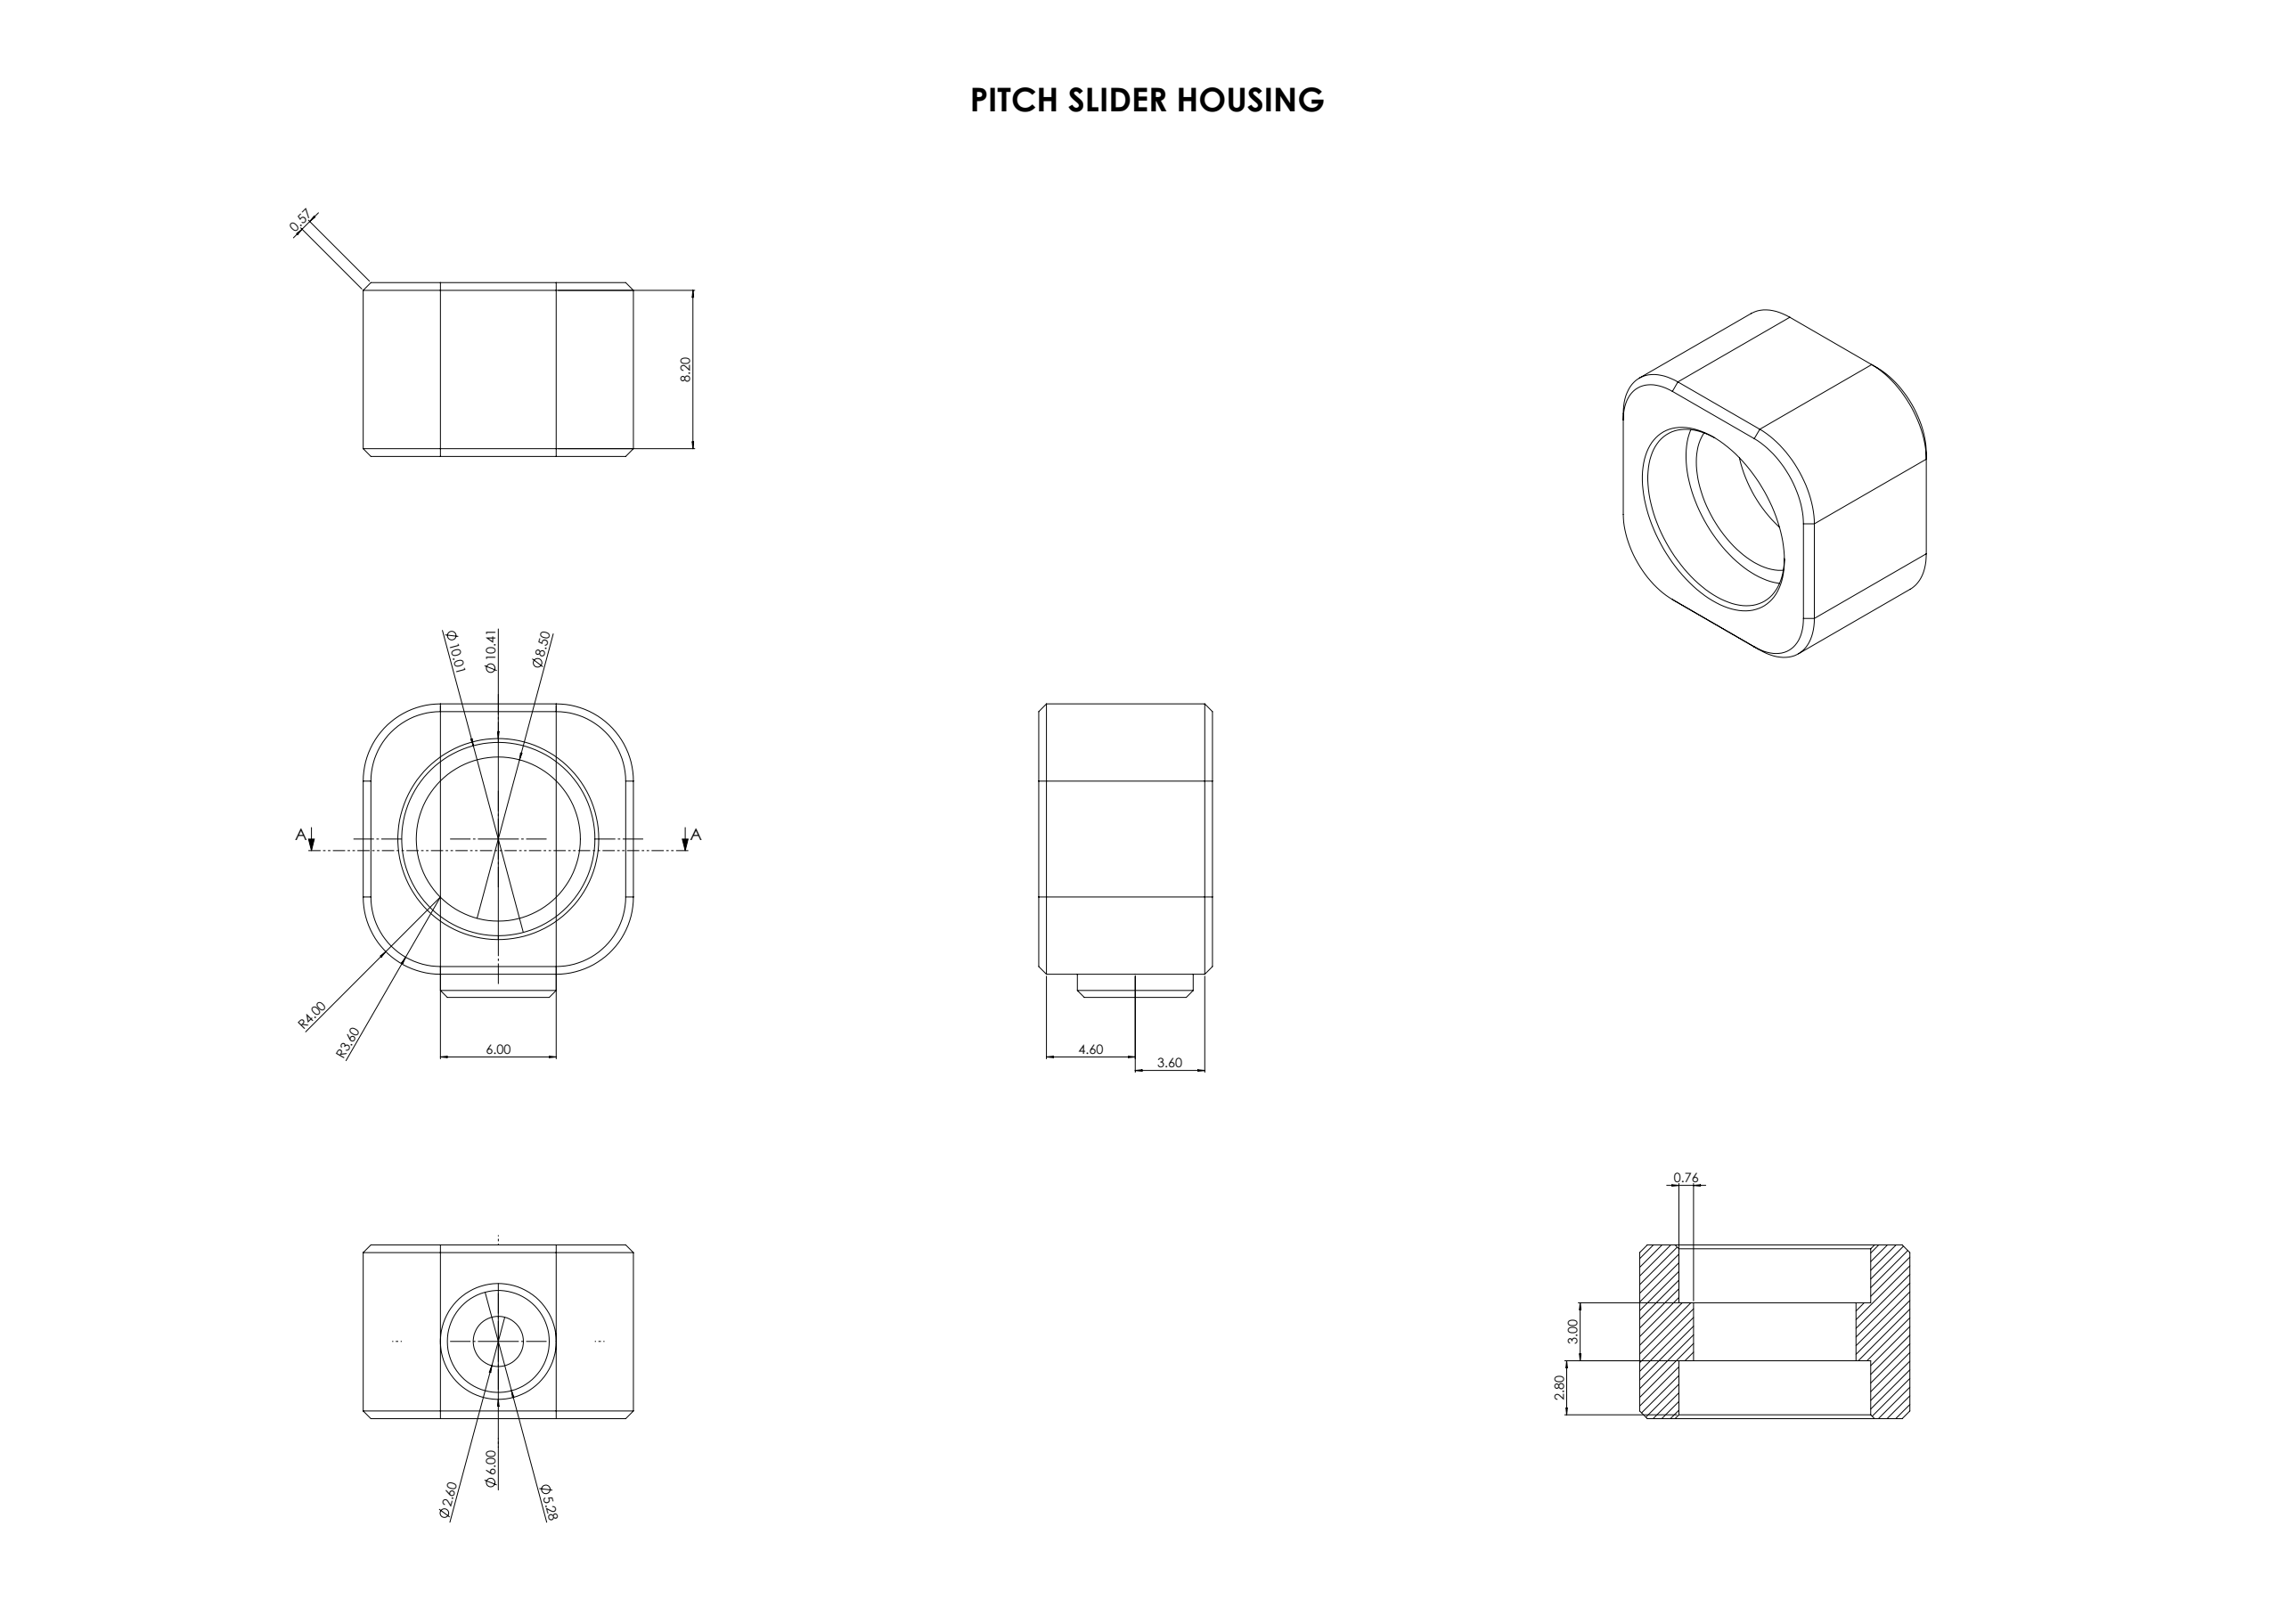
ISO-10303-21;
HEADER;
/* Generated by software containing ST-Developer
 * from STEP Tools, Inc. (www.steptools.com) 
 */

FILE_DESCRIPTION(
/* description */ (''),
/* implementation_level */ '2;1');

FILE_NAME(
/* name */ '01_Pitch_Slider_Housing.step',
/* time_stamp */ '2026-10-25T01:35:35-07:00',
/* author */ (''),
/* organization */ (''),
/* preprocessor_version */ 'ST-DEVELOPER v20.2',
/* originating_system */ 'Autodesk Translation Framework v15.15.0.0',
/* authorisation */ '');

FILE_SCHEMA (('AUTOMOTIVE_DESIGN { 1 0 10303 214 3 1 1 }'));
ENDSEC;

DATA;
#10=MECHANICAL_DESIGN_GEOMETRIC_PRESENTATION_REPRESENTATION('',(#260),#11430);
#236=SHAPE_REPRESENTATION_RELATIONSHIP('SRR','None',#11479,#248);
#248=ADVANCED_BREP_SHAPE_REPRESENTATION('',(#272),#11418);
#260=STYLED_ITEM('',(#11588),#272);
#272=MANIFOLD_SOLID_BREP('Body1',#4461);
#284=FACE_BOUND('',#797,.T.);
#285=FACE_BOUND('',#800,.T.);
#286=FACE_BOUND('',#804,.T.);
#287=FACE_BOUND('',#833,.T.);
#288=FACE_BOUND('',#836,.T.);
#323=PLANE('',#4614);
#324=PLANE('',#4619);
#325=PLANE('',#4629);
#326=PLANE('',#4636);
#327=PLANE('',#4639);
#328=PLANE('',#4642);
#329=PLANE('',#4645);
#330=PLANE('',#4650);
#331=PLANE('',#4653);
#332=PLANE('',#4654);
#333=PLANE('',#4657);
#334=PLANE('',#4660);
#335=PLANE('',#4662);
#336=PLANE('',#4665);
#337=PLANE('',#4667);
#338=PLANE('',#4670);
#339=PLANE('',#4671);
#340=PLANE('',#4675);
#341=PLANE('',#4676);
#431=CYLINDRICAL_SURFACE('',#4611,3.);
#432=CYLINDRICAL_SURFACE('',#4624,5.005);
#433=CYLINDRICAL_SURFACE('',#4634,5.005);
#434=CYLINDRICAL_SURFACE('',#4648,4.);
#435=CYLINDRICAL_SURFACE('',#4651,4.);
#436=CYLINDRICAL_SURFACE('',#4664,4.);
#437=CYLINDRICAL_SURFACE('',#4666,4.);
#438=CYLINDRICAL_SURFACE('',#4668,1.3);
#439=CYLINDRICAL_SURFACE('',#4673,4.25);
#526=FACE_OUTER_BOUND('',#794,.T.);
#527=FACE_OUTER_BOUND('',#795,.T.);
#528=FACE_OUTER_BOUND('',#796,.T.);
#529=FACE_OUTER_BOUND('',#798,.T.);
#530=FACE_OUTER_BOUND('',#799,.T.);
#531=FACE_OUTER_BOUND('',#801,.T.);
#532=FACE_OUTER_BOUND('',#802,.T.);
#533=FACE_OUTER_BOUND('',#803,.T.);
#534=FACE_OUTER_BOUND('',#805,.T.);
#535=FACE_OUTER_BOUND('',#806,.T.);
#536=FACE_OUTER_BOUND('',#807,.T.);
#537=FACE_OUTER_BOUND('',#808,.T.);
#538=FACE_OUTER_BOUND('',#809,.T.);
#539=FACE_OUTER_BOUND('',#810,.T.);
#540=FACE_OUTER_BOUND('',#811,.T.);
#541=FACE_OUTER_BOUND('',#812,.T.);
#542=FACE_OUTER_BOUND('',#813,.T.);
#543=FACE_OUTER_BOUND('',#814,.T.);
#544=FACE_OUTER_BOUND('',#815,.T.);
#545=FACE_OUTER_BOUND('',#816,.T.);
#546=FACE_OUTER_BOUND('',#817,.T.);
#547=FACE_OUTER_BOUND('',#818,.T.);
#548=FACE_OUTER_BOUND('',#819,.T.);
#549=FACE_OUTER_BOUND('',#820,.T.);
#550=FACE_OUTER_BOUND('',#821,.T.);
#551=FACE_OUTER_BOUND('',#822,.T.);
#552=FACE_OUTER_BOUND('',#823,.T.);
#553=FACE_OUTER_BOUND('',#824,.T.);
#554=FACE_OUTER_BOUND('',#825,.T.);
#555=FACE_OUTER_BOUND('',#826,.T.);
#556=FACE_OUTER_BOUND('',#827,.T.);
#557=FACE_OUTER_BOUND('',#828,.T.);
#558=FACE_OUTER_BOUND('',#829,.T.);
#559=FACE_OUTER_BOUND('',#830,.T.);
#560=FACE_OUTER_BOUND('',#831,.T.);
#561=FACE_OUTER_BOUND('',#832,.T.);
#562=FACE_OUTER_BOUND('',#834,.T.);
#563=FACE_OUTER_BOUND('',#835,.T.);
#564=FACE_OUTER_BOUND('',#837,.T.);
#794=EDGE_LOOP('',(#2885,#2886,#2887,#2888));
#795=EDGE_LOOP('',(#2889,#2890,#2891,#2892,#2893));
#796=EDGE_LOOP('',(#2894));
#797=EDGE_LOOP('',(#2895));
#798=EDGE_LOOP('',(#2896,#2897,#2898,#2899));
#799=EDGE_LOOP('',(#2900,#2901,#2902,#2903,#2904,#2905,#2906,#2907));
#800=EDGE_LOOP('',(#2908));
#801=EDGE_LOOP('',(#2909,#2910,#2911,#2912));
#802=EDGE_LOOP('',(#2913,#2914,#2915,#2916));
#803=EDGE_LOOP('',(#2917,#2918,#2919,#2920,#2921,#2922,#2923,#2924));
#804=EDGE_LOOP('',(#2925));
#805=EDGE_LOOP('',(#2926,#2927,#2928,#2929));
#806=EDGE_LOOP('',(#2930,#2931,#2932,#2933));
#807=EDGE_LOOP('',(#2934,#2935,#2936,#2937));
#808=EDGE_LOOP('',(#2938,#2939,#2940,#2941));
#809=EDGE_LOOP('',(#2942,#2943,#2944,#2945));
#810=EDGE_LOOP('',(#2946,#2947,#2948,#2949));
#811=EDGE_LOOP('',(#2950,#2951,#2952,#2953));
#812=EDGE_LOOP('',(#2954,#2955,#2956,#2957));
#813=EDGE_LOOP('',(#2958,#2959,#2960,#2961));
#814=EDGE_LOOP('',(#2962,#2963,#2964,#2965));
#815=EDGE_LOOP('',(#2966,#2967,#2968,#2969));
#816=EDGE_LOOP('',(#2970,#2971,#2972,#2973,#2974));
#817=EDGE_LOOP('',(#2975,#2976,#2977,#2978));
#818=EDGE_LOOP('',(#2979,#2980,#2981,#2982));
#819=EDGE_LOOP('',(#2983,#2984,#2985,#2986));
#820=EDGE_LOOP('',(#2987,#2988,#2989,#2990));
#821=EDGE_LOOP('',(#2991,#2992,#2993,#2994));
#822=EDGE_LOOP('',(#2995,#2996,#2997,#2998));
#823=EDGE_LOOP('',(#2999,#3000,#3001,#3002));
#824=EDGE_LOOP('',(#3003,#3004,#3005,#3006));
#825=EDGE_LOOP('',(#3007,#3008,#3009,#3010));
#826=EDGE_LOOP('',(#3011,#3012,#3013,#3014));
#827=EDGE_LOOP('',(#3015,#3016,#3017,#3018));
#828=EDGE_LOOP('',(#3019,#3020,#3021,#3022,#3023));
#829=EDGE_LOOP('',(#3024,#3025,#3026,#3027));
#830=EDGE_LOOP('',(#3028,#3029,#3030,#3031));
#831=EDGE_LOOP('',(#3032));
#832=EDGE_LOOP('',(#3033));
#833=EDGE_LOOP('',(#3034));
#834=EDGE_LOOP('',(#3035,#3036,#3037,#3038));
#835=EDGE_LOOP('',(#3039));
#836=EDGE_LOOP('',(#3040));
#837=EDGE_LOOP('',(#3041,#3042,#3043,#3044));
#1101=LINE('',#6333,#1391);
#1102=LINE('',#6337,#1392);
#1103=LINE('',#6348,#1393);
#1104=LINE('',#6353,#1394);
#1105=LINE('',#6357,#1395);
#1106=LINE('',#6361,#1396);
#1107=LINE('',#6365,#1397);
#1108=LINE('',#6370,#1398);
#1109=LINE('',#6375,#1399);
#1110=LINE('',#6380,#1400);
#1111=LINE('',#6384,#1401);
#1112=LINE('',#6388,#1402);
#1113=LINE('',#6392,#1403);
#1114=LINE('',#6396,#1404);
#1115=LINE('',#6400,#1405);
#1116=LINE('',#6402,#1406);
#1117=LINE('',#6403,#1407);
#1118=LINE('',#6406,#1408);
#1119=LINE('',#6410,#1409);
#1120=LINE('',#6411,#1410);
#1121=LINE('',#6414,#1411);
#1122=LINE('',#6418,#1412);
#1123=LINE('',#6419,#1413);
#1124=LINE('',#6422,#1414);
#1125=LINE('',#6426,#1415);
#1126=LINE('',#6427,#1416);
#1127=LINE('',#6432,#1417);
#1128=LINE('',#6435,#1418);
#1129=LINE('',#6438,#1419);
#1130=LINE('',#6439,#1420);
#1131=LINE('',#6441,#1421);
#1132=LINE('',#6443,#1422);
#1133=LINE('',#6446,#1423);
#1134=LINE('',#6449,#1424);
#1135=LINE('',#6450,#1425);
#1136=LINE('',#6451,#1426);
#1137=LINE('',#6454,#1427);
#1138=LINE('',#6458,#1428);
#1139=LINE('',#6459,#1429);
#1140=LINE('',#6462,#1430);
#1141=LINE('',#6465,#1431);
#1142=LINE('',#6466,#1432);
#1143=LINE('',#6468,#1433);
#1144=LINE('',#6470,#1434);
#1145=LINE('',#6473,#1435);
#1146=LINE('',#6474,#1436);
#1147=LINE('',#6476,#1437);
#1148=LINE('',#6478,#1438);
#1149=LINE('',#6482,#1439);
#1150=LINE('',#6490,#1440);
#1391=VECTOR('',#5091,2.82);
#1392=VECTOR('',#5096,3.);
#1393=VECTOR('',#5109,5.105);
#1394=VECTOR('',#5114,10.);
#1395=VECTOR('',#5117,10.);
#1396=VECTOR('',#5120,10.);
#1397=VECTOR('',#5123,10.);
#1398=VECTOR('',#5130,5.005);
#1399=VECTOR('',#5135,5.105);
#1400=VECTOR('',#5140,10.);
#1401=VECTOR('',#5143,10.);
#1402=VECTOR('',#5146,10.);
#1403=VECTOR('',#5149,10.);
#1404=VECTOR('',#5154,5.005);
#1405=VECTOR('',#5159,10.);
#1406=VECTOR('',#5160,10.);
#1407=VECTOR('',#5161,10.);
#1408=VECTOR('',#5164,10.);
#1409=VECTOR('',#5169,10.);
#1410=VECTOR('',#5170,10.);
#1411=VECTOR('',#5173,10.);
#1412=VECTOR('',#5178,10.);
#1413=VECTOR('',#5179,10.);
#1414=VECTOR('',#5182,10.);
#1415=VECTOR('',#5187,10.);
#1416=VECTOR('',#5188,10.);
#1417=VECTOR('',#5195,10.);
#1418=VECTOR('',#5198,10.);
#1419=VECTOR('',#5201,10.);
#1420=VECTOR('',#5202,10.);
#1421=VECTOR('',#5205,10.);
#1422=VECTOR('',#5206,10.);
#1423=VECTOR('',#5211,10.);
#1424=VECTOR('',#5214,10.);
#1425=VECTOR('',#5215,10.);
#1426=VECTOR('',#5216,10.);
#1427=VECTOR('',#5219,10.);
#1428=VECTOR('',#5224,10.);
#1429=VECTOR('',#5225,10.);
#1430=VECTOR('',#5228,10.);
#1431=VECTOR('',#5233,10.);
#1432=VECTOR('',#5234,10.);
#1433=VECTOR('',#5237,10.);
#1434=VECTOR('',#5240,10.);
#1435=VECTOR('',#5245,10.);
#1436=VECTOR('',#5246,10.);
#1437=VECTOR('',#5249,10.);
#1438=VECTOR('',#5252,10.);
#1439=VECTOR('',#5257,1.3);
#1440=VECTOR('',#5268,4.25);
#1681=CIRCLE('',#4609,2.64);
#1682=CIRCLE('',#4610,3.);
#1683=CIRCLE('',#4612,3.);
#1684=CIRCLE('',#4613,3.);
#1685=CIRCLE('',#4615,1.3);
#1686=CIRCLE('',#4617,5.205);
#1687=CIRCLE('',#4618,5.005);
#1688=CIRCLE('',#4620,3.6);
#1689=CIRCLE('',#4621,3.6);
#1690=CIRCLE('',#4622,3.6);
#1691=CIRCLE('',#4623,3.6);
#1692=CIRCLE('',#4625,5.005);
#1693=CIRCLE('',#4627,5.205);
#1694=CIRCLE('',#4628,5.005);
#1695=CIRCLE('',#4630,3.6);
#1696=CIRCLE('',#4631,3.6);
#1697=CIRCLE('',#4632,3.6);
#1698=CIRCLE('',#4633,3.6);
#1699=CIRCLE('',#4635,5.005);
#1700=CIRCLE('',#4638,4.);
#1701=CIRCLE('',#4641,4.);
#1702=CIRCLE('',#4644,4.);
#1703=CIRCLE('',#4647,4.);
#1704=CIRCLE('',#4649,4.);
#1705=CIRCLE('',#4652,4.);
#1706=CIRCLE('',#4656,4.);
#1707=CIRCLE('',#4659,4.);
#1708=CIRCLE('',#4669,1.3);
#1709=CIRCLE('',#4672,4.25);
#1710=CIRCLE('',#4674,4.25);
#1866=VERTEX_POINT('',#6330);
#1867=VERTEX_POINT('',#6332);
#1868=VERTEX_POINT('',#6336);
#1869=VERTEX_POINT('',#6338);
#1870=VERTEX_POINT('',#6342);
#1871=VERTEX_POINT('',#6345);
#1872=VERTEX_POINT('',#6347);
#1873=VERTEX_POINT('',#6351);
#1874=VERTEX_POINT('',#6352);
#1875=VERTEX_POINT('',#6354);
#1876=VERTEX_POINT('',#6356);
#1877=VERTEX_POINT('',#6358);
#1878=VERTEX_POINT('',#6360);
#1879=VERTEX_POINT('',#6362);
#1880=VERTEX_POINT('',#6364);
#1881=VERTEX_POINT('',#6368);
#1882=VERTEX_POINT('',#6372);
#1883=VERTEX_POINT('',#6374);
#1884=VERTEX_POINT('',#6378);
#1885=VERTEX_POINT('',#6379);
#1886=VERTEX_POINT('',#6381);
#1887=VERTEX_POINT('',#6383);
#1888=VERTEX_POINT('',#6385);
#1889=VERTEX_POINT('',#6387);
#1890=VERTEX_POINT('',#6389);
#1891=VERTEX_POINT('',#6391);
#1892=VERTEX_POINT('',#6395);
#1893=VERTEX_POINT('',#6399);
#1894=VERTEX_POINT('',#6401);
#1895=VERTEX_POINT('',#6405);
#1896=VERTEX_POINT('',#6409);
#1897=VERTEX_POINT('',#6413);
#1898=VERTEX_POINT('',#6417);
#1899=VERTEX_POINT('',#6421);
#1900=VERTEX_POINT('',#6425);
#1901=VERTEX_POINT('',#6431);
#1902=VERTEX_POINT('',#6433);
#1903=VERTEX_POINT('',#6437);
#1904=VERTEX_POINT('',#6442);
#1905=VERTEX_POINT('',#6448);
#1906=VERTEX_POINT('',#6453);
#1907=VERTEX_POINT('',#6457);
#1908=VERTEX_POINT('',#6461);
#1909=VERTEX_POINT('',#6481);
#1910=VERTEX_POINT('',#6486);
#1911=VERTEX_POINT('',#6489);
#2260=EDGE_CURVE('',#1866,#1866,#1681,.T.);
#2261=EDGE_CURVE('',#1866,#1867,#1101,.T.);
#2262=EDGE_CURVE('',#1867,#1867,#1682,.T.);
#2263=EDGE_CURVE('',#1867,#1868,#1102,.T.);
#2264=EDGE_CURVE('',#1869,#1868,#1683,.T.);
#2265=EDGE_CURVE('',#1868,#1869,#1684,.T.);
#2266=EDGE_CURVE('',#1870,#1870,#1685,.T.);
#2267=EDGE_CURVE('',#1871,#1871,#1686,.T.);
#2268=EDGE_CURVE('',#1871,#1872,#1103,.T.);
#2269=EDGE_CURVE('',#1872,#1872,#1687,.T.);
#2270=EDGE_CURVE('',#1873,#1874,#1104,.T.);
#2271=EDGE_CURVE('',#1875,#1873,#1688,.T.);
#2272=EDGE_CURVE('',#1876,#1875,#1105,.T.);
#2273=EDGE_CURVE('',#1877,#1876,#1689,.T.);
#2274=EDGE_CURVE('',#1878,#1877,#1106,.T.);
#2275=EDGE_CURVE('',#1879,#1878,#1690,.T.);
#2276=EDGE_CURVE('',#1880,#1879,#1107,.T.);
#2277=EDGE_CURVE('',#1874,#1880,#1691,.T.);
#2278=EDGE_CURVE('',#1881,#1881,#1692,.T.);
#2279=EDGE_CURVE('',#1881,#1872,#1108,.T.);
#2280=EDGE_CURVE('',#1882,#1882,#1693,.T.);
#2281=EDGE_CURVE('',#1882,#1883,#1109,.T.);
#2282=EDGE_CURVE('',#1883,#1883,#1694,.T.);
#2283=EDGE_CURVE('',#1884,#1885,#1110,.T.);
#2284=EDGE_CURVE('',#1886,#1884,#1695,.T.);
#2285=EDGE_CURVE('',#1887,#1886,#1111,.T.);
#2286=EDGE_CURVE('',#1888,#1887,#1696,.T.);
#2287=EDGE_CURVE('',#1889,#1888,#1112,.T.);
#2288=EDGE_CURVE('',#1890,#1889,#1697,.T.);
#2289=EDGE_CURVE('',#1891,#1890,#1113,.T.);
#2290=EDGE_CURVE('',#1885,#1891,#1698,.T.);
#2291=EDGE_CURVE('',#1883,#1892,#1114,.T.);
#2292=EDGE_CURVE('',#1892,#1892,#1699,.T.);
#2293=EDGE_CURVE('',#1885,#1893,#1115,.T.);
#2294=EDGE_CURVE('',#1893,#1894,#1116,.T.);
#2295=EDGE_CURVE('',#1894,#1884,#1117,.T.);
#2296=EDGE_CURVE('',#1891,#1895,#1118,.T.);
#2297=EDGE_CURVE('',#1895,#1893,#1700,.T.);
#2298=EDGE_CURVE('',#1890,#1896,#1119,.T.);
#2299=EDGE_CURVE('',#1896,#1895,#1120,.T.);
#2300=EDGE_CURVE('',#1889,#1897,#1121,.T.);
#2301=EDGE_CURVE('',#1897,#1896,#1701,.T.);
#2302=EDGE_CURVE('',#1888,#1898,#1122,.T.);
#2303=EDGE_CURVE('',#1898,#1897,#1123,.T.);
#2304=EDGE_CURVE('',#1887,#1899,#1124,.T.);
#2305=EDGE_CURVE('',#1899,#1898,#1702,.T.);
#2306=EDGE_CURVE('',#1886,#1900,#1125,.T.);
#2307=EDGE_CURVE('',#1900,#1899,#1126,.T.);
#2308=EDGE_CURVE('',#1894,#1900,#1703,.T.);
#2309=EDGE_CURVE('',#1899,#1901,#1127,.T.);
#2310=EDGE_CURVE('',#1902,#1901,#1704,.T.);
#2311=EDGE_CURVE('',#1898,#1902,#1128,.T.);
#2312=EDGE_CURVE('',#1900,#1903,#1129,.T.);
#2313=EDGE_CURVE('',#1901,#1903,#1130,.T.);
#2314=EDGE_CURVE('',#1894,#1868,#1131,.T.);
#2315=EDGE_CURVE('',#1868,#1904,#1132,.T.);
#2316=EDGE_CURVE('',#1903,#1904,#1705,.T.);
#2317=EDGE_CURVE('',#1893,#1869,#1133,.T.);
#2318=EDGE_CURVE('',#1905,#1873,#1134,.T.);
#2319=EDGE_CURVE('',#1874,#1904,#1135,.T.);
#2320=EDGE_CURVE('',#1904,#1905,#1136,.T.);
#2321=EDGE_CURVE('',#1906,#1875,#1137,.T.);
#2322=EDGE_CURVE('',#1905,#1906,#1706,.T.);
#2323=EDGE_CURVE('',#1907,#1876,#1138,.T.);
#2324=EDGE_CURVE('',#1906,#1907,#1139,.T.);
#2325=EDGE_CURVE('',#1908,#1877,#1140,.T.);
#2326=EDGE_CURVE('',#1907,#1908,#1707,.T.);
#2327=EDGE_CURVE('',#1902,#1878,#1141,.T.);
#2328=EDGE_CURVE('',#1908,#1902,#1142,.T.);
#2329=EDGE_CURVE('',#1901,#1879,#1143,.T.);
#2330=EDGE_CURVE('',#1903,#1880,#1144,.T.);
#2331=EDGE_CURVE('',#1897,#1908,#1145,.T.);
#2332=EDGE_CURVE('',#1896,#1907,#1146,.T.);
#2333=EDGE_CURVE('',#1895,#1906,#1147,.T.);
#2334=EDGE_CURVE('',#1869,#1905,#1148,.T.);
#2335=EDGE_CURVE('',#1870,#1909,#1149,.T.);
#2336=EDGE_CURVE('',#1909,#1909,#1708,.T.);
#2337=EDGE_CURVE('',#1910,#1910,#1709,.T.);
#2338=EDGE_CURVE('',#1910,#1911,#1150,.T.);
#2339=EDGE_CURVE('',#1911,#1911,#1710,.T.);
#2885=ORIENTED_EDGE('',*,*,#2260,.T.);
#2886=ORIENTED_EDGE('',*,*,#2261,.T.);
#2887=ORIENTED_EDGE('',*,*,#2262,.T.);
#2888=ORIENTED_EDGE('',*,*,#2261,.F.);
#2889=ORIENTED_EDGE('',*,*,#2262,.F.);
#2890=ORIENTED_EDGE('',*,*,#2263,.T.);
#2891=ORIENTED_EDGE('',*,*,#2264,.F.);
#2892=ORIENTED_EDGE('',*,*,#2265,.F.);
#2893=ORIENTED_EDGE('',*,*,#2263,.F.);
#2894=ORIENTED_EDGE('',*,*,#2260,.F.);
#2895=ORIENTED_EDGE('',*,*,#2266,.T.);
#2896=ORIENTED_EDGE('',*,*,#2267,.T.);
#2897=ORIENTED_EDGE('',*,*,#2268,.T.);
#2898=ORIENTED_EDGE('',*,*,#2269,.T.);
#2899=ORIENTED_EDGE('',*,*,#2268,.F.);
#2900=ORIENTED_EDGE('',*,*,#2270,.F.);
#2901=ORIENTED_EDGE('',*,*,#2271,.F.);
#2902=ORIENTED_EDGE('',*,*,#2272,.F.);
#2903=ORIENTED_EDGE('',*,*,#2273,.F.);
#2904=ORIENTED_EDGE('',*,*,#2274,.F.);
#2905=ORIENTED_EDGE('',*,*,#2275,.F.);
#2906=ORIENTED_EDGE('',*,*,#2276,.F.);
#2907=ORIENTED_EDGE('',*,*,#2277,.F.);
#2908=ORIENTED_EDGE('',*,*,#2267,.F.);
#2909=ORIENTED_EDGE('',*,*,#2278,.F.);
#2910=ORIENTED_EDGE('',*,*,#2279,.T.);
#2911=ORIENTED_EDGE('',*,*,#2269,.F.);
#2912=ORIENTED_EDGE('',*,*,#2279,.F.);
#2913=ORIENTED_EDGE('',*,*,#2280,.T.);
#2914=ORIENTED_EDGE('',*,*,#2281,.T.);
#2915=ORIENTED_EDGE('',*,*,#2282,.T.);
#2916=ORIENTED_EDGE('',*,*,#2281,.F.);
#2917=ORIENTED_EDGE('',*,*,#2283,.F.);
#2918=ORIENTED_EDGE('',*,*,#2284,.F.);
#2919=ORIENTED_EDGE('',*,*,#2285,.F.);
#2920=ORIENTED_EDGE('',*,*,#2286,.F.);
#2921=ORIENTED_EDGE('',*,*,#2287,.F.);
#2922=ORIENTED_EDGE('',*,*,#2288,.F.);
#2923=ORIENTED_EDGE('',*,*,#2289,.F.);
#2924=ORIENTED_EDGE('',*,*,#2290,.F.);
#2925=ORIENTED_EDGE('',*,*,#2280,.F.);
#2926=ORIENTED_EDGE('',*,*,#2282,.F.);
#2927=ORIENTED_EDGE('',*,*,#2291,.T.);
#2928=ORIENTED_EDGE('',*,*,#2292,.T.);
#2929=ORIENTED_EDGE('',*,*,#2291,.F.);
#2930=ORIENTED_EDGE('',*,*,#2293,.T.);
#2931=ORIENTED_EDGE('',*,*,#2294,.T.);
#2932=ORIENTED_EDGE('',*,*,#2295,.T.);
#2933=ORIENTED_EDGE('',*,*,#2283,.T.);
#2934=ORIENTED_EDGE('',*,*,#2296,.T.);
#2935=ORIENTED_EDGE('',*,*,#2297,.T.);
#2936=ORIENTED_EDGE('',*,*,#2293,.F.);
#2937=ORIENTED_EDGE('',*,*,#2290,.T.);
#2938=ORIENTED_EDGE('',*,*,#2298,.T.);
#2939=ORIENTED_EDGE('',*,*,#2299,.T.);
#2940=ORIENTED_EDGE('',*,*,#2296,.F.);
#2941=ORIENTED_EDGE('',*,*,#2289,.T.);
#2942=ORIENTED_EDGE('',*,*,#2300,.T.);
#2943=ORIENTED_EDGE('',*,*,#2301,.T.);
#2944=ORIENTED_EDGE('',*,*,#2298,.F.);
#2945=ORIENTED_EDGE('',*,*,#2288,.T.);
#2946=ORIENTED_EDGE('',*,*,#2302,.T.);
#2947=ORIENTED_EDGE('',*,*,#2303,.T.);
#2948=ORIENTED_EDGE('',*,*,#2300,.F.);
#2949=ORIENTED_EDGE('',*,*,#2287,.T.);
#2950=ORIENTED_EDGE('',*,*,#2304,.T.);
#2951=ORIENTED_EDGE('',*,*,#2305,.T.);
#2952=ORIENTED_EDGE('',*,*,#2302,.F.);
#2953=ORIENTED_EDGE('',*,*,#2286,.T.);
#2954=ORIENTED_EDGE('',*,*,#2306,.T.);
#2955=ORIENTED_EDGE('',*,*,#2307,.T.);
#2956=ORIENTED_EDGE('',*,*,#2304,.F.);
#2957=ORIENTED_EDGE('',*,*,#2285,.T.);
#2958=ORIENTED_EDGE('',*,*,#2295,.F.);
#2959=ORIENTED_EDGE('',*,*,#2308,.T.);
#2960=ORIENTED_EDGE('',*,*,#2306,.F.);
#2961=ORIENTED_EDGE('',*,*,#2284,.T.);
#2962=ORIENTED_EDGE('',*,*,#2305,.F.);
#2963=ORIENTED_EDGE('',*,*,#2309,.T.);
#2964=ORIENTED_EDGE('',*,*,#2310,.F.);
#2965=ORIENTED_EDGE('',*,*,#2311,.F.);
#2966=ORIENTED_EDGE('',*,*,#2307,.F.);
#2967=ORIENTED_EDGE('',*,*,#2312,.T.);
#2968=ORIENTED_EDGE('',*,*,#2313,.F.);
#2969=ORIENTED_EDGE('',*,*,#2309,.F.);
#2970=ORIENTED_EDGE('',*,*,#2308,.F.);
#2971=ORIENTED_EDGE('',*,*,#2314,.T.);
#2972=ORIENTED_EDGE('',*,*,#2315,.T.);
#2973=ORIENTED_EDGE('',*,*,#2316,.F.);
#2974=ORIENTED_EDGE('',*,*,#2312,.F.);
#2975=ORIENTED_EDGE('',*,*,#2294,.F.);
#2976=ORIENTED_EDGE('',*,*,#2317,.T.);
#2977=ORIENTED_EDGE('',*,*,#2264,.T.);
#2978=ORIENTED_EDGE('',*,*,#2314,.F.);
#2979=ORIENTED_EDGE('',*,*,#2318,.T.);
#2980=ORIENTED_EDGE('',*,*,#2270,.T.);
#2981=ORIENTED_EDGE('',*,*,#2319,.T.);
#2982=ORIENTED_EDGE('',*,*,#2320,.T.);
#2983=ORIENTED_EDGE('',*,*,#2321,.T.);
#2984=ORIENTED_EDGE('',*,*,#2271,.T.);
#2985=ORIENTED_EDGE('',*,*,#2318,.F.);
#2986=ORIENTED_EDGE('',*,*,#2322,.T.);
#2987=ORIENTED_EDGE('',*,*,#2323,.T.);
#2988=ORIENTED_EDGE('',*,*,#2272,.T.);
#2989=ORIENTED_EDGE('',*,*,#2321,.F.);
#2990=ORIENTED_EDGE('',*,*,#2324,.T.);
#2991=ORIENTED_EDGE('',*,*,#2325,.T.);
#2992=ORIENTED_EDGE('',*,*,#2273,.T.);
#2993=ORIENTED_EDGE('',*,*,#2323,.F.);
#2994=ORIENTED_EDGE('',*,*,#2326,.T.);
#2995=ORIENTED_EDGE('',*,*,#2327,.T.);
#2996=ORIENTED_EDGE('',*,*,#2274,.T.);
#2997=ORIENTED_EDGE('',*,*,#2325,.F.);
#2998=ORIENTED_EDGE('',*,*,#2328,.T.);
#2999=ORIENTED_EDGE('',*,*,#2329,.T.);
#3000=ORIENTED_EDGE('',*,*,#2275,.T.);
#3001=ORIENTED_EDGE('',*,*,#2327,.F.);
#3002=ORIENTED_EDGE('',*,*,#2310,.T.);
#3003=ORIENTED_EDGE('',*,*,#2330,.T.);
#3004=ORIENTED_EDGE('',*,*,#2276,.T.);
#3005=ORIENTED_EDGE('',*,*,#2329,.F.);
#3006=ORIENTED_EDGE('',*,*,#2313,.T.);
#3007=ORIENTED_EDGE('',*,*,#2319,.F.);
#3008=ORIENTED_EDGE('',*,*,#2277,.T.);
#3009=ORIENTED_EDGE('',*,*,#2330,.F.);
#3010=ORIENTED_EDGE('',*,*,#2316,.T.);
#3011=ORIENTED_EDGE('',*,*,#2301,.F.);
#3012=ORIENTED_EDGE('',*,*,#2331,.T.);
#3013=ORIENTED_EDGE('',*,*,#2326,.F.);
#3014=ORIENTED_EDGE('',*,*,#2332,.F.);
#3015=ORIENTED_EDGE('',*,*,#2299,.F.);
#3016=ORIENTED_EDGE('',*,*,#2332,.T.);
#3017=ORIENTED_EDGE('',*,*,#2324,.F.);
#3018=ORIENTED_EDGE('',*,*,#2333,.F.);
#3019=ORIENTED_EDGE('',*,*,#2297,.F.);
#3020=ORIENTED_EDGE('',*,*,#2333,.T.);
#3021=ORIENTED_EDGE('',*,*,#2322,.F.);
#3022=ORIENTED_EDGE('',*,*,#2334,.F.);
#3023=ORIENTED_EDGE('',*,*,#2317,.F.);
#3024=ORIENTED_EDGE('',*,*,#2320,.F.);
#3025=ORIENTED_EDGE('',*,*,#2315,.F.);
#3026=ORIENTED_EDGE('',*,*,#2265,.T.);
#3027=ORIENTED_EDGE('',*,*,#2334,.T.);
#3028=ORIENTED_EDGE('',*,*,#2266,.F.);
#3029=ORIENTED_EDGE('',*,*,#2335,.T.);
#3030=ORIENTED_EDGE('',*,*,#2336,.T.);
#3031=ORIENTED_EDGE('',*,*,#2335,.F.);
#3032=ORIENTED_EDGE('',*,*,#2336,.F.);
#3033=ORIENTED_EDGE('',*,*,#2292,.F.);
#3034=ORIENTED_EDGE('',*,*,#2337,.T.);
#3035=ORIENTED_EDGE('',*,*,#2337,.F.);
#3036=ORIENTED_EDGE('',*,*,#2338,.T.);
#3037=ORIENTED_EDGE('',*,*,#2339,.T.);
#3038=ORIENTED_EDGE('',*,*,#2338,.F.);
#3039=ORIENTED_EDGE('',*,*,#2278,.T.);
#3040=ORIENTED_EDGE('',*,*,#2339,.F.);
#3041=ORIENTED_EDGE('',*,*,#2303,.F.);
#3042=ORIENTED_EDGE('',*,*,#2311,.T.);
#3043=ORIENTED_EDGE('',*,*,#2328,.F.);
#3044=ORIENTED_EDGE('',*,*,#2331,.F.);
#4135=CONICAL_SURFACE('',#4608,2.82,0.785398163397448);
#4136=CONICAL_SURFACE('',#4616,5.105,0.785398163397448);
#4137=CONICAL_SURFACE('',#4626,5.105,0.785398163397448);
#4138=CONICAL_SURFACE('',#4637,3.8,0.785398163397449);
#4139=CONICAL_SURFACE('',#4640,3.8,0.785398163397449);
#4140=CONICAL_SURFACE('',#4643,3.8,0.785398163397449);
#4141=CONICAL_SURFACE('',#4646,3.8,0.785398163397449);
#4142=CONICAL_SURFACE('',#4655,3.8,0.785398163397448);
#4143=CONICAL_SURFACE('',#4658,3.8,0.785398163397448);
#4144=CONICAL_SURFACE('',#4661,3.8,0.785398163397448);
#4145=CONICAL_SURFACE('',#4663,3.8,0.785398163397448);
#4193=ADVANCED_FACE('',(#526),#4135,.T.);
#4194=ADVANCED_FACE('',(#527),#431,.T.);
#4195=ADVANCED_FACE('',(#528,#284),#323,.F.);
#4196=ADVANCED_FACE('',(#529),#4136,.F.);
#4197=ADVANCED_FACE('',(#530,#285),#324,.T.);
#4198=ADVANCED_FACE('',(#531),#432,.F.);
#4199=ADVANCED_FACE('',(#532),#4137,.F.);
#4200=ADVANCED_FACE('',(#533,#286),#325,.F.);
#4201=ADVANCED_FACE('',(#534),#433,.F.);
#4202=ADVANCED_FACE('',(#535),#326,.T.);
#4203=ADVANCED_FACE('',(#536),#4138,.T.);
#4204=ADVANCED_FACE('',(#537),#327,.T.);
#4205=ADVANCED_FACE('',(#538),#4139,.T.);
#4206=ADVANCED_FACE('',(#539),#328,.T.);
#4207=ADVANCED_FACE('',(#540),#4140,.T.);
#4208=ADVANCED_FACE('',(#541),#329,.T.);
#4209=ADVANCED_FACE('',(#542),#4141,.T.);
#4210=ADVANCED_FACE('',(#543),#434,.T.);
#4211=ADVANCED_FACE('',(#544),#330,.T.);
#4212=ADVANCED_FACE('',(#545),#435,.T.);
#4213=ADVANCED_FACE('',(#546),#331,.T.);
#4214=ADVANCED_FACE('',(#547),#332,.T.);
#4215=ADVANCED_FACE('',(#548),#4142,.T.);
#4216=ADVANCED_FACE('',(#549),#333,.T.);
#4217=ADVANCED_FACE('',(#550),#4143,.T.);
#4218=ADVANCED_FACE('',(#551),#334,.T.);
#4219=ADVANCED_FACE('',(#552),#4144,.T.);
#4220=ADVANCED_FACE('',(#553),#335,.T.);
#4221=ADVANCED_FACE('',(#554),#4145,.T.);
#4222=ADVANCED_FACE('',(#555),#436,.T.);
#4223=ADVANCED_FACE('',(#556),#336,.T.);
#4224=ADVANCED_FACE('',(#557),#437,.T.);
#4225=ADVANCED_FACE('',(#558),#337,.T.);
#4226=ADVANCED_FACE('',(#559),#438,.F.);
#4227=ADVANCED_FACE('',(#560),#338,.F.);
#4228=ADVANCED_FACE('',(#561,#287),#339,.F.);
#4229=ADVANCED_FACE('',(#562),#439,.F.);
#4230=ADVANCED_FACE('',(#563,#288),#340,.F.);
#4231=ADVANCED_FACE('',(#564),#341,.T.);
#4461=CLOSED_SHELL('',(#4193,#4194,#4195,#4196,#4197,#4198,#4199,#4200,
#4201,#4202,#4203,#4204,#4205,#4206,#4207,#4208,#4209,#4210,#4211,#4212,
#4213,#4214,#4215,#4216,#4217,#4218,#4219,#4220,#4221,#4222,#4223,#4224,
#4225,#4226,#4227,#4228,#4229,#4230,#4231));
#4607=AXIS2_PLACEMENT_3D('',#6328,#5085,#5086);
#4608=AXIS2_PLACEMENT_3D('',#6329,#5087,#5088);
#4609=AXIS2_PLACEMENT_3D('',#6331,#5089,#5090);
#4610=AXIS2_PLACEMENT_3D('',#6334,#5092,#5093);
#4611=AXIS2_PLACEMENT_3D('',#6335,#5094,#5095);
#4612=AXIS2_PLACEMENT_3D('',#6339,#5097,#5098);
#4613=AXIS2_PLACEMENT_3D('',#6340,#5099,#5100);
#4614=AXIS2_PLACEMENT_3D('',#6341,#5101,#5102);
#4615=AXIS2_PLACEMENT_3D('',#6343,#5103,#5104);
#4616=AXIS2_PLACEMENT_3D('',#6344,#5105,#5106);
#4617=AXIS2_PLACEMENT_3D('',#6346,#5107,#5108);
#4618=AXIS2_PLACEMENT_3D('',#6349,#5110,#5111);
#4619=AXIS2_PLACEMENT_3D('',#6350,#5112,#5113);
#4620=AXIS2_PLACEMENT_3D('',#6355,#5115,#5116);
#4621=AXIS2_PLACEMENT_3D('',#6359,#5118,#5119);
#4622=AXIS2_PLACEMENT_3D('',#6363,#5121,#5122);
#4623=AXIS2_PLACEMENT_3D('',#6366,#5124,#5125);
#4624=AXIS2_PLACEMENT_3D('',#6367,#5126,#5127);
#4625=AXIS2_PLACEMENT_3D('',#6369,#5128,#5129);
#4626=AXIS2_PLACEMENT_3D('',#6371,#5131,#5132);
#4627=AXIS2_PLACEMENT_3D('',#6373,#5133,#5134);
#4628=AXIS2_PLACEMENT_3D('',#6376,#5136,#5137);
#4629=AXIS2_PLACEMENT_3D('',#6377,#5138,#5139);
#4630=AXIS2_PLACEMENT_3D('',#6382,#5141,#5142);
#4631=AXIS2_PLACEMENT_3D('',#6386,#5144,#5145);
#4632=AXIS2_PLACEMENT_3D('',#6390,#5147,#5148);
#4633=AXIS2_PLACEMENT_3D('',#6393,#5150,#5151);
#4634=AXIS2_PLACEMENT_3D('',#6394,#5152,#5153);
#4635=AXIS2_PLACEMENT_3D('',#6397,#5155,#5156);
#4636=AXIS2_PLACEMENT_3D('',#6398,#5157,#5158);
#4637=AXIS2_PLACEMENT_3D('',#6404,#5162,#5163);
#4638=AXIS2_PLACEMENT_3D('',#6407,#5165,#5166);
#4639=AXIS2_PLACEMENT_3D('',#6408,#5167,#5168);
#4640=AXIS2_PLACEMENT_3D('',#6412,#5171,#5172);
#4641=AXIS2_PLACEMENT_3D('',#6415,#5174,#5175);
#4642=AXIS2_PLACEMENT_3D('',#6416,#5176,#5177);
#4643=AXIS2_PLACEMENT_3D('',#6420,#5180,#5181);
#4644=AXIS2_PLACEMENT_3D('',#6423,#5183,#5184);
#4645=AXIS2_PLACEMENT_3D('',#6424,#5185,#5186);
#4646=AXIS2_PLACEMENT_3D('',#6428,#5189,#5190);
#4647=AXIS2_PLACEMENT_3D('',#6429,#5191,#5192);
#4648=AXIS2_PLACEMENT_3D('',#6430,#5193,#5194);
#4649=AXIS2_PLACEMENT_3D('',#6434,#5196,#5197);
#4650=AXIS2_PLACEMENT_3D('',#6436,#5199,#5200);
#4651=AXIS2_PLACEMENT_3D('',#6440,#5203,#5204);
#4652=AXIS2_PLACEMENT_3D('',#6444,#5207,#5208);
#4653=AXIS2_PLACEMENT_3D('',#6445,#5209,#5210);
#4654=AXIS2_PLACEMENT_3D('',#6447,#5212,#5213);
#4655=AXIS2_PLACEMENT_3D('',#6452,#5217,#5218);
#4656=AXIS2_PLACEMENT_3D('',#6455,#5220,#5221);
#4657=AXIS2_PLACEMENT_3D('',#6456,#5222,#5223);
#4658=AXIS2_PLACEMENT_3D('',#6460,#5226,#5227);
#4659=AXIS2_PLACEMENT_3D('',#6463,#5229,#5230);
#4660=AXIS2_PLACEMENT_3D('',#6464,#5231,#5232);
#4661=AXIS2_PLACEMENT_3D('',#6467,#5235,#5236);
#4662=AXIS2_PLACEMENT_3D('',#6469,#5238,#5239);
#4663=AXIS2_PLACEMENT_3D('',#6471,#5241,#5242);
#4664=AXIS2_PLACEMENT_3D('',#6472,#5243,#5244);
#4665=AXIS2_PLACEMENT_3D('',#6475,#5247,#5248);
#4666=AXIS2_PLACEMENT_3D('',#6477,#5250,#5251);
#4667=AXIS2_PLACEMENT_3D('',#6479,#5253,#5254);
#4668=AXIS2_PLACEMENT_3D('',#6480,#5255,#5256);
#4669=AXIS2_PLACEMENT_3D('',#6483,#5258,#5259);
#4670=AXIS2_PLACEMENT_3D('',#6484,#5260,#5261);
#4671=AXIS2_PLACEMENT_3D('',#6485,#5262,#5263);
#4672=AXIS2_PLACEMENT_3D('',#6487,#5264,#5265);
#4673=AXIS2_PLACEMENT_3D('',#6488,#5266,#5267);
#4674=AXIS2_PLACEMENT_3D('',#6491,#5269,#5270);
#4675=AXIS2_PLACEMENT_3D('',#6492,#5271,#5272);
#4676=AXIS2_PLACEMENT_3D('',#6493,#5273,#5274);
#5085=DIRECTION('axis',(0.,0.,1.));
#5086=DIRECTION('refdir',(1.,0.,0.));
#5087=DIRECTION('center_axis',(0.,1.,0.));
#5088=DIRECTION('ref_axis',(1.,0.,0.));
#5089=DIRECTION('center_axis',(0.,1.,0.));
#5090=DIRECTION('ref_axis',(1.,0.,0.));
#5091=DIRECTION('',(-0.707106781186547,0.707106781186548,-8.65956056235493E-17));
#5092=DIRECTION('center_axis',(0.,-1.,0.));
#5093=DIRECTION('ref_axis',(1.,0.,0.));
#5094=DIRECTION('center_axis',(0.,-1.,0.));
#5095=DIRECTION('ref_axis',(1.,0.,0.));
#5096=DIRECTION('',(0.,1.,0.));
#5097=DIRECTION('center_axis',(0.,1.,0.));
#5098=DIRECTION('ref_axis',(1.,0.,0.));
#5099=DIRECTION('center_axis',(0.,1.,0.));
#5100=DIRECTION('ref_axis',(1.,0.,0.));
#5101=DIRECTION('center_axis',(0.,1.,0.));
#5102=DIRECTION('ref_axis',(1.,0.,0.));
#5103=DIRECTION('center_axis',(0.,1.,0.));
#5104=DIRECTION('ref_axis',(1.,0.,0.));
#5105=DIRECTION('center_axis',(0.,0.,1.));
#5106=DIRECTION('ref_axis',(1.,0.,0.));
#5107=DIRECTION('center_axis',(0.,0.,1.));
#5108=DIRECTION('ref_axis',(1.,0.,0.));
#5109=DIRECTION('',(0.707106781186548,8.65956056235493E-17,-0.707106781186548));
#5110=DIRECTION('center_axis',(0.,0.,-1.));
#5111=DIRECTION('ref_axis',(1.,0.,0.));
#5112=DIRECTION('center_axis',(0.,0.,1.));
#5113=DIRECTION('ref_axis',(1.,0.,0.));
#5114=DIRECTION('',(-1.,0.,0.));
#5115=DIRECTION('center_axis',(0.,0.,-1.));
#5116=DIRECTION('ref_axis',(0.,-1.,0.));
#5117=DIRECTION('',(0.,-1.,0.));
#5118=DIRECTION('center_axis',(0.,0.,-1.));
#5119=DIRECTION('ref_axis',(1.,0.,0.));
#5120=DIRECTION('',(1.,0.,0.));
#5121=DIRECTION('center_axis',(0.,0.,-1.));
#5122=DIRECTION('ref_axis',(0.,1.,0.));
#5123=DIRECTION('',(0.,1.,0.));
#5124=DIRECTION('center_axis',(0.,0.,-1.));
#5125=DIRECTION('ref_axis',(-1.,0.,0.));
#5126=DIRECTION('center_axis',(0.,0.,1.));
#5127=DIRECTION('ref_axis',(1.,0.,0.));
#5128=DIRECTION('center_axis',(0.,0.,1.));
#5129=DIRECTION('ref_axis',(1.,0.,0.));
#5130=DIRECTION('',(0.,0.,1.));
#5131=DIRECTION('center_axis',(0.,0.,-1.));
#5132=DIRECTION('ref_axis',(1.,0.,0.));
#5133=DIRECTION('center_axis',(0.,0.,-1.));
#5134=DIRECTION('ref_axis',(1.,0.,0.));
#5135=DIRECTION('',(0.707106781186548,-8.65956056235493E-17,0.707106781186548));
#5136=DIRECTION('center_axis',(0.,0.,1.));
#5137=DIRECTION('ref_axis',(1.,0.,0.));
#5138=DIRECTION('center_axis',(0.,0.,1.));
#5139=DIRECTION('ref_axis',(1.,0.,0.));
#5140=DIRECTION('',(1.,0.,0.));
#5141=DIRECTION('center_axis',(0.,0.,1.));
#5142=DIRECTION('ref_axis',(-1.,0.,0.));
#5143=DIRECTION('',(0.,-1.,0.));
#5144=DIRECTION('center_axis',(0.,0.,1.));
#5145=DIRECTION('ref_axis',(0.,1.,0.));
#5146=DIRECTION('',(-1.,0.,0.));
#5147=DIRECTION('center_axis',(0.,0.,1.));
#5148=DIRECTION('ref_axis',(1.,0.,0.));
#5149=DIRECTION('',(0.,1.,0.));
#5150=DIRECTION('center_axis',(0.,0.,1.));
#5151=DIRECTION('ref_axis',(0.,-1.,0.));
#5152=DIRECTION('center_axis',(0.,0.,1.));
#5153=DIRECTION('ref_axis',(1.,0.,0.));
#5154=DIRECTION('',(0.,0.,1.));
#5155=DIRECTION('center_axis',(0.,0.,1.));
#5156=DIRECTION('ref_axis',(1.,0.,0.));
#5157=DIRECTION('center_axis',(0.,-0.707106781186547,-0.707106781186548));
#5158=DIRECTION('ref_axis',(-1.,0.,0.));
#5159=DIRECTION('',(0.,-0.707106781186548,0.707106781186547));
#5160=DIRECTION('',(-1.,0.,0.));
#5161=DIRECTION('',(0.,0.707106781186548,-0.707106781186547));
#5162=DIRECTION('center_axis',(0.,0.,1.));
#5163=DIRECTION('ref_axis',(0.,-1.,0.));
#5164=DIRECTION('',(0.707106781186548,0.,0.707106781186547));
#5165=DIRECTION('center_axis',(0.,0.,-1.));
#5166=DIRECTION('ref_axis',(0.,-1.,0.));
#5167=DIRECTION('center_axis',(0.707106781186547,0.,-0.707106781186548));
#5168=DIRECTION('ref_axis',(-0.707106781186548,0.,-0.707106781186547));
#5169=DIRECTION('',(0.707106781186548,0.,0.707106781186547));
#5170=DIRECTION('',(0.,-1.,0.));
#5171=DIRECTION('center_axis',(0.,0.,1.));
#5172=DIRECTION('ref_axis',(1.,0.,0.));
#5173=DIRECTION('',(0.,0.707106781186548,0.707106781186547));
#5174=DIRECTION('center_axis',(0.,0.,-1.));
#5175=DIRECTION('ref_axis',(1.,0.,0.));
#5176=DIRECTION('center_axis',(0.,0.707106781186547,-0.707106781186548));
#5177=DIRECTION('ref_axis',(-1.,0.,0.));
#5178=DIRECTION('',(0.,0.707106781186548,0.707106781186547));
#5179=DIRECTION('',(1.,0.,0.));
#5180=DIRECTION('center_axis',(0.,0.,1.));
#5181=DIRECTION('ref_axis',(0.,1.,0.));
#5182=DIRECTION('',(-0.707106781186548,0.,0.707106781186547));
#5183=DIRECTION('center_axis',(0.,0.,-1.));
#5184=DIRECTION('ref_axis',(0.,1.,0.));
#5185=DIRECTION('center_axis',(-0.707106781186547,0.,-0.707106781186548));
#5186=DIRECTION('ref_axis',(-0.707106781186548,0.,0.707106781186547));
#5187=DIRECTION('',(-0.707106781186548,0.,0.707106781186547));
#5188=DIRECTION('',(0.,1.,0.));
#5189=DIRECTION('center_axis',(0.,0.,1.));
#5190=DIRECTION('ref_axis',(-1.,0.,0.));
#5191=DIRECTION('center_axis',(0.,0.,-1.));
#5192=DIRECTION('ref_axis',(-1.,0.,0.));
#5193=DIRECTION('center_axis',(0.,0.,1.));
#5194=DIRECTION('ref_axis',(0.,1.,0.));
#5195=DIRECTION('',(0.,0.,1.));
#5196=DIRECTION('center_axis',(0.,0.,1.));
#5197=DIRECTION('ref_axis',(0.,1.,0.));
#5198=DIRECTION('',(0.,0.,1.));
#5199=DIRECTION('center_axis',(-1.,0.,0.));
#5200=DIRECTION('ref_axis',(0.,-1.,0.));
#5201=DIRECTION('',(0.,0.,1.));
#5202=DIRECTION('',(0.,-1.,0.));
#5203=DIRECTION('center_axis',(0.,0.,1.));
#5204=DIRECTION('ref_axis',(-1.,0.,0.));
#5205=DIRECTION('',(0.,0.,1.));
#5206=DIRECTION('',(0.,0.,1.));
#5207=DIRECTION('center_axis',(0.,0.,1.));
#5208=DIRECTION('ref_axis',(-1.,0.,0.));
#5209=DIRECTION('center_axis',(0.,-1.,0.));
#5210=DIRECTION('ref_axis',(1.,0.,0.));
#5211=DIRECTION('',(0.,0.,1.));
#5212=DIRECTION('center_axis',(0.,-0.707106781186548,0.707106781186548));
#5213=DIRECTION('ref_axis',(1.,0.,0.));
#5214=DIRECTION('',(0.,0.707106781186548,0.707106781186548));
#5215=DIRECTION('',(0.,-0.707106781186548,-0.707106781186548));
#5216=DIRECTION('',(1.,0.,0.));
#5217=DIRECTION('center_axis',(0.,0.,-1.));
#5218=DIRECTION('ref_axis',(0.,-1.,0.));
#5219=DIRECTION('',(-0.707106781186548,0.,0.707106781186548));
#5220=DIRECTION('center_axis',(0.,0.,1.));
#5221=DIRECTION('ref_axis',(0.,-1.,0.));
#5222=DIRECTION('center_axis',(0.707106781186548,0.,0.707106781186548));
#5223=DIRECTION('ref_axis',(0.707106781186548,0.,-0.707106781186548));
#5224=DIRECTION('',(-0.707106781186548,0.,0.707106781186548));
#5225=DIRECTION('',(0.,1.,0.));
#5226=DIRECTION('center_axis',(0.,0.,-1.));
#5227=DIRECTION('ref_axis',(1.,0.,0.));
#5228=DIRECTION('',(0.,-0.707106781186548,0.707106781186548));
#5229=DIRECTION('center_axis',(0.,0.,1.));
#5230=DIRECTION('ref_axis',(1.,0.,0.));
#5231=DIRECTION('center_axis',(0.,0.707106781186548,0.707106781186548));
#5232=DIRECTION('ref_axis',(1.,0.,0.));
#5233=DIRECTION('',(0.,-0.707106781186548,0.707106781186548));
#5234=DIRECTION('',(-1.,0.,0.));
#5235=DIRECTION('center_axis',(0.,0.,-1.));
#5236=DIRECTION('ref_axis',(0.,1.,0.));
#5237=DIRECTION('',(0.707106781186548,0.,0.707106781186548));
#5238=DIRECTION('center_axis',(-0.707106781186548,0.,0.707106781186548));
#5239=DIRECTION('ref_axis',(0.707106781186548,0.,0.707106781186548));
#5240=DIRECTION('',(0.707106781186548,0.,0.707106781186548));
#5241=DIRECTION('center_axis',(0.,0.,-1.));
#5242=DIRECTION('ref_axis',(-1.,0.,0.));
#5243=DIRECTION('center_axis',(0.,0.,1.));
#5244=DIRECTION('ref_axis',(1.,0.,0.));
#5245=DIRECTION('',(0.,0.,1.));
#5246=DIRECTION('',(0.,0.,1.));
#5247=DIRECTION('center_axis',(1.,0.,0.));
#5248=DIRECTION('ref_axis',(0.,1.,0.));
#5249=DIRECTION('',(0.,0.,1.));
#5250=DIRECTION('center_axis',(0.,0.,1.));
#5251=DIRECTION('ref_axis',(0.,-1.,0.));
#5252=DIRECTION('',(0.,0.,1.));
#5253=DIRECTION('center_axis',(0.,-1.,0.));
#5254=DIRECTION('ref_axis',(1.,0.,0.));
#5255=DIRECTION('center_axis',(0.,1.,0.));
#5256=DIRECTION('ref_axis',(1.,0.,0.));
#5257=DIRECTION('',(0.,1.,0.));
#5258=DIRECTION('center_axis',(0.,1.,0.));
#5259=DIRECTION('ref_axis',(1.,0.,0.));
#5260=DIRECTION('center_axis',(0.,1.,0.));
#5261=DIRECTION('ref_axis',(1.,0.,0.));
#5262=DIRECTION('center_axis',(0.,0.,1.));
#5263=DIRECTION('ref_axis',(1.,0.,0.));
#5264=DIRECTION('center_axis',(0.,0.,1.));
#5265=DIRECTION('ref_axis',(1.,0.,0.));
#5266=DIRECTION('center_axis',(0.,0.,1.));
#5267=DIRECTION('ref_axis',(1.,0.,0.));
#5268=DIRECTION('',(0.,0.,1.));
#5269=DIRECTION('center_axis',(0.,0.,1.));
#5270=DIRECTION('ref_axis',(1.,0.,0.));
#5271=DIRECTION('center_axis',(0.,0.,-1.));
#5272=DIRECTION('ref_axis',(-1.,0.,0.));
#5273=DIRECTION('center_axis',(0.,1.,0.));
#5274=DIRECTION('ref_axis',(-1.,0.,0.));
#6328=CARTESIAN_POINT('',(0.,0.,0.));
#6329=CARTESIAN_POINT('Origin',(0.,-8.02,4.));
#6330=CARTESIAN_POINT('',(-2.64,-8.2,4.));
#6331=CARTESIAN_POINT('Origin',(0.,-8.2,4.));
#6332=CARTESIAN_POINT('',(-3.,-7.84,4.));
#6333=CARTESIAN_POINT('',(-2.82,-8.02,4.));
#6334=CARTESIAN_POINT('Origin',(0.,-7.84,4.));
#6335=CARTESIAN_POINT('Origin',(0.,-7.,4.));
#6336=CARTESIAN_POINT('',(-3.,-7.,4.));
#6337=CARTESIAN_POINT('',(-3.,-7.,4.));
#6338=CARTESIAN_POINT('',(3.,-7.,4.));
#6339=CARTESIAN_POINT('Origin',(0.,-7.,4.));
#6340=CARTESIAN_POINT('Origin',(0.,-7.,4.));
#6341=CARTESIAN_POINT('Origin',(0.,-8.2,4.));
#6342=CARTESIAN_POINT('',(-1.3,-8.2,4.));
#6343=CARTESIAN_POINT('Origin',(0.,-8.2,4.));
#6344=CARTESIAN_POINT('Origin',(0.,0.,8.9));
#6345=CARTESIAN_POINT('',(-5.205,-6.37428658956197E-16,9.));
#6346=CARTESIAN_POINT('Origin',(0.,0.,9.));
#6347=CARTESIAN_POINT('',(-5.005,6.1293572297325E-16,8.8));
#6348=CARTESIAN_POINT('',(-5.105,-6.25182190964724E-16,8.9));
#6349=CARTESIAN_POINT('Origin',(0.,0.,8.8));
#6350=CARTESIAN_POINT('Origin',(0.,0.,9.));
#6351=CARTESIAN_POINT('',(3.,-6.6,9.));
#6352=CARTESIAN_POINT('',(-3.,-6.6,9.));
#6353=CARTESIAN_POINT('',(-1.5,-6.6,9.));
#6354=CARTESIAN_POINT('',(6.6,-3.,9.));
#6355=CARTESIAN_POINT('Origin',(3.,-3.,9.));
#6356=CARTESIAN_POINT('',(6.6,3.,9.));
#6357=CARTESIAN_POINT('',(6.6,-1.5,9.));
#6358=CARTESIAN_POINT('',(3.,6.6,9.));
#6359=CARTESIAN_POINT('Origin',(3.,3.,9.));
#6360=CARTESIAN_POINT('',(-3.,6.6,9.));
#6361=CARTESIAN_POINT('',(1.5,6.6,9.));
#6362=CARTESIAN_POINT('',(-6.6,3.,9.));
#6363=CARTESIAN_POINT('Origin',(-3.,3.,9.));
#6364=CARTESIAN_POINT('',(-6.6,-3.,9.));
#6365=CARTESIAN_POINT('',(-6.6,1.5,9.));
#6366=CARTESIAN_POINT('Origin',(-3.,-3.,9.));
#6367=CARTESIAN_POINT('Origin',(0.,0.,7.55));
#6368=CARTESIAN_POINT('',(-5.005,-6.1293572297325E-16,6.));
#6369=CARTESIAN_POINT('Origin',(0.,0.,6.));
#6370=CARTESIAN_POINT('',(-5.005,-6.1293572297325E-16,7.55));
#6371=CARTESIAN_POINT('Origin',(0.,0.,0.1));
#6372=CARTESIAN_POINT('',(-5.205,6.37428658956197E-16,0.));
#6373=CARTESIAN_POINT('Origin',(0.,0.,0.));
#6374=CARTESIAN_POINT('',(-5.005,-6.1293572297325E-16,0.2));
#6375=CARTESIAN_POINT('',(-5.105,6.25182190964724E-16,0.1));
#6376=CARTESIAN_POINT('Origin',(0.,0.,0.2));
#6377=CARTESIAN_POINT('Origin',(0.,0.,0.));
#6378=CARTESIAN_POINT('',(-3.,-6.6,0.));
#6379=CARTESIAN_POINT('',(3.,-6.6,0.));
#6380=CARTESIAN_POINT('',(-1.5,-6.6,0.));
#6381=CARTESIAN_POINT('',(-6.6,-3.,0.));
#6382=CARTESIAN_POINT('Origin',(-3.,-3.,0.));
#6383=CARTESIAN_POINT('',(-6.6,3.,0.));
#6384=CARTESIAN_POINT('',(-6.6,1.5,0.));
#6385=CARTESIAN_POINT('',(-3.,6.6,0.));
#6386=CARTESIAN_POINT('Origin',(-3.,3.,0.));
#6387=CARTESIAN_POINT('',(3.,6.6,0.));
#6388=CARTESIAN_POINT('',(1.5,6.6,0.));
#6389=CARTESIAN_POINT('',(6.6,3.,0.));
#6390=CARTESIAN_POINT('Origin',(3.,3.,0.));
#6391=CARTESIAN_POINT('',(6.6,-3.,0.));
#6392=CARTESIAN_POINT('',(6.6,-1.5,0.));
#6393=CARTESIAN_POINT('Origin',(3.,-3.,0.));
#6394=CARTESIAN_POINT('Origin',(0.,0.,1.45));
#6395=CARTESIAN_POINT('',(-5.005,-6.1293572297325E-16,3.));
#6396=CARTESIAN_POINT('',(-5.005,-6.1293572297325E-16,1.45));
#6397=CARTESIAN_POINT('Origin',(0.,0.,3.));
#6398=CARTESIAN_POINT('Origin',(-1.5,-6.8,0.2));
#6399=CARTESIAN_POINT('',(3.,-7.,0.4));
#6400=CARTESIAN_POINT('',(3.,-6.6,0.));
#6401=CARTESIAN_POINT('',(-3.,-7.,0.4));
#6402=CARTESIAN_POINT('',(-1.5,-7.,0.4));
#6403=CARTESIAN_POINT('',(-3.,-7.,0.4));
#6404=CARTESIAN_POINT('Origin',(3.,-3.,0.2));
#6405=CARTESIAN_POINT('',(7.,-3.,0.4));
#6406=CARTESIAN_POINT('',(6.6,-3.,0.));
#6407=CARTESIAN_POINT('Origin',(3.,-3.,0.4));
#6408=CARTESIAN_POINT('Origin',(6.8,-1.5,0.2));
#6409=CARTESIAN_POINT('',(7.,3.,0.4));
#6410=CARTESIAN_POINT('',(6.6,3.,0.));
#6411=CARTESIAN_POINT('',(7.,-1.5,0.4));
#6412=CARTESIAN_POINT('Origin',(3.,3.,0.2));
#6413=CARTESIAN_POINT('',(3.,7.,0.4));
#6414=CARTESIAN_POINT('',(3.,6.6,0.));
#6415=CARTESIAN_POINT('Origin',(3.,3.,0.4));
#6416=CARTESIAN_POINT('Origin',(1.5,6.8,0.2));
#6417=CARTESIAN_POINT('',(-3.,7.,0.4));
#6418=CARTESIAN_POINT('',(-3.,6.6,0.));
#6419=CARTESIAN_POINT('',(1.5,7.,0.4));
#6420=CARTESIAN_POINT('Origin',(-3.,3.,0.2));
#6421=CARTESIAN_POINT('',(-7.,3.,0.4));
#6422=CARTESIAN_POINT('',(-6.6,3.,0.));
#6423=CARTESIAN_POINT('Origin',(-3.,3.,0.4));
#6424=CARTESIAN_POINT('Origin',(-6.8,1.5,0.2));
#6425=CARTESIAN_POINT('',(-7.,-3.,0.4));
#6426=CARTESIAN_POINT('',(-6.6,-3.,0.));
#6427=CARTESIAN_POINT('',(-7.,1.5,0.4));
#6428=CARTESIAN_POINT('Origin',(-3.,-3.,0.2));
#6429=CARTESIAN_POINT('Origin',(-3.,-3.,0.4));
#6430=CARTESIAN_POINT('Origin',(-3.,3.,0.));
#6431=CARTESIAN_POINT('',(-7.,3.,8.6));
#6432=CARTESIAN_POINT('',(-7.,3.,0.));
#6433=CARTESIAN_POINT('',(-3.,7.,8.6));
#6434=CARTESIAN_POINT('Origin',(-3.,3.,8.6));
#6435=CARTESIAN_POINT('',(-3.,7.,0.));
#6436=CARTESIAN_POINT('Origin',(-7.,3.,0.));
#6437=CARTESIAN_POINT('',(-7.,-3.,8.6));
#6438=CARTESIAN_POINT('',(-7.,-3.,0.));
#6439=CARTESIAN_POINT('',(-7.,1.5,8.6));
#6440=CARTESIAN_POINT('Origin',(-3.,-3.,0.));
#6441=CARTESIAN_POINT('',(-3.,-7.,0.));
#6442=CARTESIAN_POINT('',(-3.,-7.,8.6));
#6443=CARTESIAN_POINT('',(-3.,-7.,0.));
#6444=CARTESIAN_POINT('Origin',(-3.,-3.,8.6));
#6445=CARTESIAN_POINT('Origin',(-3.,-7.,0.));
#6446=CARTESIAN_POINT('',(3.,-7.,0.));
#6447=CARTESIAN_POINT('Origin',(-1.5,-6.8,8.8));
#6448=CARTESIAN_POINT('',(3.,-7.,8.6));
#6449=CARTESIAN_POINT('',(3.,-7.,8.6));
#6450=CARTESIAN_POINT('',(-3.,-6.6,9.));
#6451=CARTESIAN_POINT('',(-1.5,-7.,8.6));
#6452=CARTESIAN_POINT('Origin',(3.,-3.,8.8));
#6453=CARTESIAN_POINT('',(7.,-3.,8.6));
#6454=CARTESIAN_POINT('',(7.,-3.,8.6));
#6455=CARTESIAN_POINT('Origin',(3.,-3.,8.6));
#6456=CARTESIAN_POINT('Origin',(6.8,-1.5,8.8));
#6457=CARTESIAN_POINT('',(7.,3.,8.6));
#6458=CARTESIAN_POINT('',(7.,3.,8.6));
#6459=CARTESIAN_POINT('',(7.,-1.5,8.6));
#6460=CARTESIAN_POINT('Origin',(3.,3.,8.8));
#6461=CARTESIAN_POINT('',(3.,7.,8.6));
#6462=CARTESIAN_POINT('',(3.,7.,8.6));
#6463=CARTESIAN_POINT('Origin',(3.,3.,8.6));
#6464=CARTESIAN_POINT('Origin',(1.5,6.8,8.8));
#6465=CARTESIAN_POINT('',(-3.,7.,8.6));
#6466=CARTESIAN_POINT('',(1.5,7.,8.6));
#6467=CARTESIAN_POINT('Origin',(-3.,3.,8.8));
#6468=CARTESIAN_POINT('',(-7.,3.,8.6));
#6469=CARTESIAN_POINT('Origin',(-6.8,1.5,8.8));
#6470=CARTESIAN_POINT('',(-7.,-3.,8.6));
#6471=CARTESIAN_POINT('Origin',(-3.,-3.,8.8));
#6472=CARTESIAN_POINT('Origin',(3.,3.,0.));
#6473=CARTESIAN_POINT('',(3.,7.,0.));
#6474=CARTESIAN_POINT('',(7.,3.,0.));
#6475=CARTESIAN_POINT('Origin',(7.,-3.,0.));
#6476=CARTESIAN_POINT('',(7.,-3.,0.));
#6477=CARTESIAN_POINT('Origin',(3.,-3.,0.));
#6478=CARTESIAN_POINT('',(3.,-7.,0.));
#6479=CARTESIAN_POINT('Origin',(-3.,-7.,0.));
#6480=CARTESIAN_POINT('Origin',(0.,-8.2,4.));
#6481=CARTESIAN_POINT('',(-1.3,-5.6,4.));
#6482=CARTESIAN_POINT('',(-1.3,-8.2,4.));
#6483=CARTESIAN_POINT('Origin',(0.,-5.6,4.));
#6484=CARTESIAN_POINT('Origin',(0.,-5.6,4.));
#6485=CARTESIAN_POINT('Origin',(4.25,0.,3.));
#6486=CARTESIAN_POINT('',(-4.25,-5.20474889637625E-16,3.));
#6487=CARTESIAN_POINT('Origin',(0.,0.,3.));
#6488=CARTESIAN_POINT('Origin',(0.,0.,4.5));
#6489=CARTESIAN_POINT('',(-4.25,-5.20474889637625E-16,6.));
#6490=CARTESIAN_POINT('',(-4.25,-5.20474889637625E-16,4.5));
#6491=CARTESIAN_POINT('Origin',(0.,0.,6.));
#6492=CARTESIAN_POINT('Origin',(5.005,0.,6.));
#6493=CARTESIAN_POINT('Origin',(3.,7.,0.));
#11404=UNCERTAINTY_MEASURE_WITH_UNIT(LENGTH_MEASURE(0.01),#11431,
'DISTANCE_ACCURACY_VALUE',
'Maximum model space distance between geometric entities at asserted c
onnectivities');
#11416=UNCERTAINTY_MEASURE_WITH_UNIT(LENGTH_MEASURE(0.01),#11431,
'DISTANCE_ACCURACY_VALUE',
'Maximum model space distance between geometric entities at asserted c
onnectivities');
#11418=(
GEOMETRIC_REPRESENTATION_CONTEXT(3)
GLOBAL_UNCERTAINTY_ASSIGNED_CONTEXT((#11404))
GLOBAL_UNIT_ASSIGNED_CONTEXT((#11431,#11433,#11434))
REPRESENTATION_CONTEXT('','3D')
);
#11430=(
GEOMETRIC_REPRESENTATION_CONTEXT(3)
GLOBAL_UNCERTAINTY_ASSIGNED_CONTEXT((#11416))
GLOBAL_UNIT_ASSIGNED_CONTEXT((#11431,#11433,#11434))
REPRESENTATION_CONTEXT('','3D')
);
#11431=(
LENGTH_UNIT()
NAMED_UNIT(*)
SI_UNIT(.MILLI.,.METRE.)
);
#11433=(
NAMED_UNIT(*)
PLANE_ANGLE_UNIT()
SI_UNIT($,.RADIAN.)
);
#11434=(
NAMED_UNIT(*)
SI_UNIT($,.STERADIAN.)
SOLID_ANGLE_UNIT()
);
#11436=SHAPE_DEFINITION_REPRESENTATION(#11449,#11479);
#11449=PRODUCT_DEFINITION_SHAPE('',$,#11493);
#11479=SHAPE_REPRESENTATION('',(#4607),#11418);
#11491=PRODUCT_DEFINITION_CONTEXT('part definition',#11532,'design');
#11493=PRODUCT_DEFINITION('2026-10-25-00-55-37-066',
'01_Pitch_Slider_Housing',#11506,#11491);
#11506=PRODUCT_DEFINITION_FORMATION('',$,#11535);
#11532=APPLICATION_CONTEXT(
'Core Data for Automotive Mechanical Design Process');
#11533=PRODUCT_CONTEXT('part definition',#11532,'mechanical');
#11535=PRODUCT('2026-10-25-00-55-37-066','01_Pitch_Slider_Housing',$,(#11533));
#11582=COLOUR_RGB('Dark Blue',0.08,0.2,0.34);
#11583=FILL_AREA_STYLE_COLOUR('',#11582);
#11584=FILL_AREA_STYLE('',(#11583));
#11585=SURFACE_STYLE_FILL_AREA(#11584);
#11586=SURFACE_SIDE_STYLE('',(#11585));
#11587=SURFACE_STYLE_USAGE(.BOTH.,#11586);
#11588=PRESENTATION_STYLE_ASSIGNMENT((#11587));
ENDSEC;
END-ISO-10303-21;
